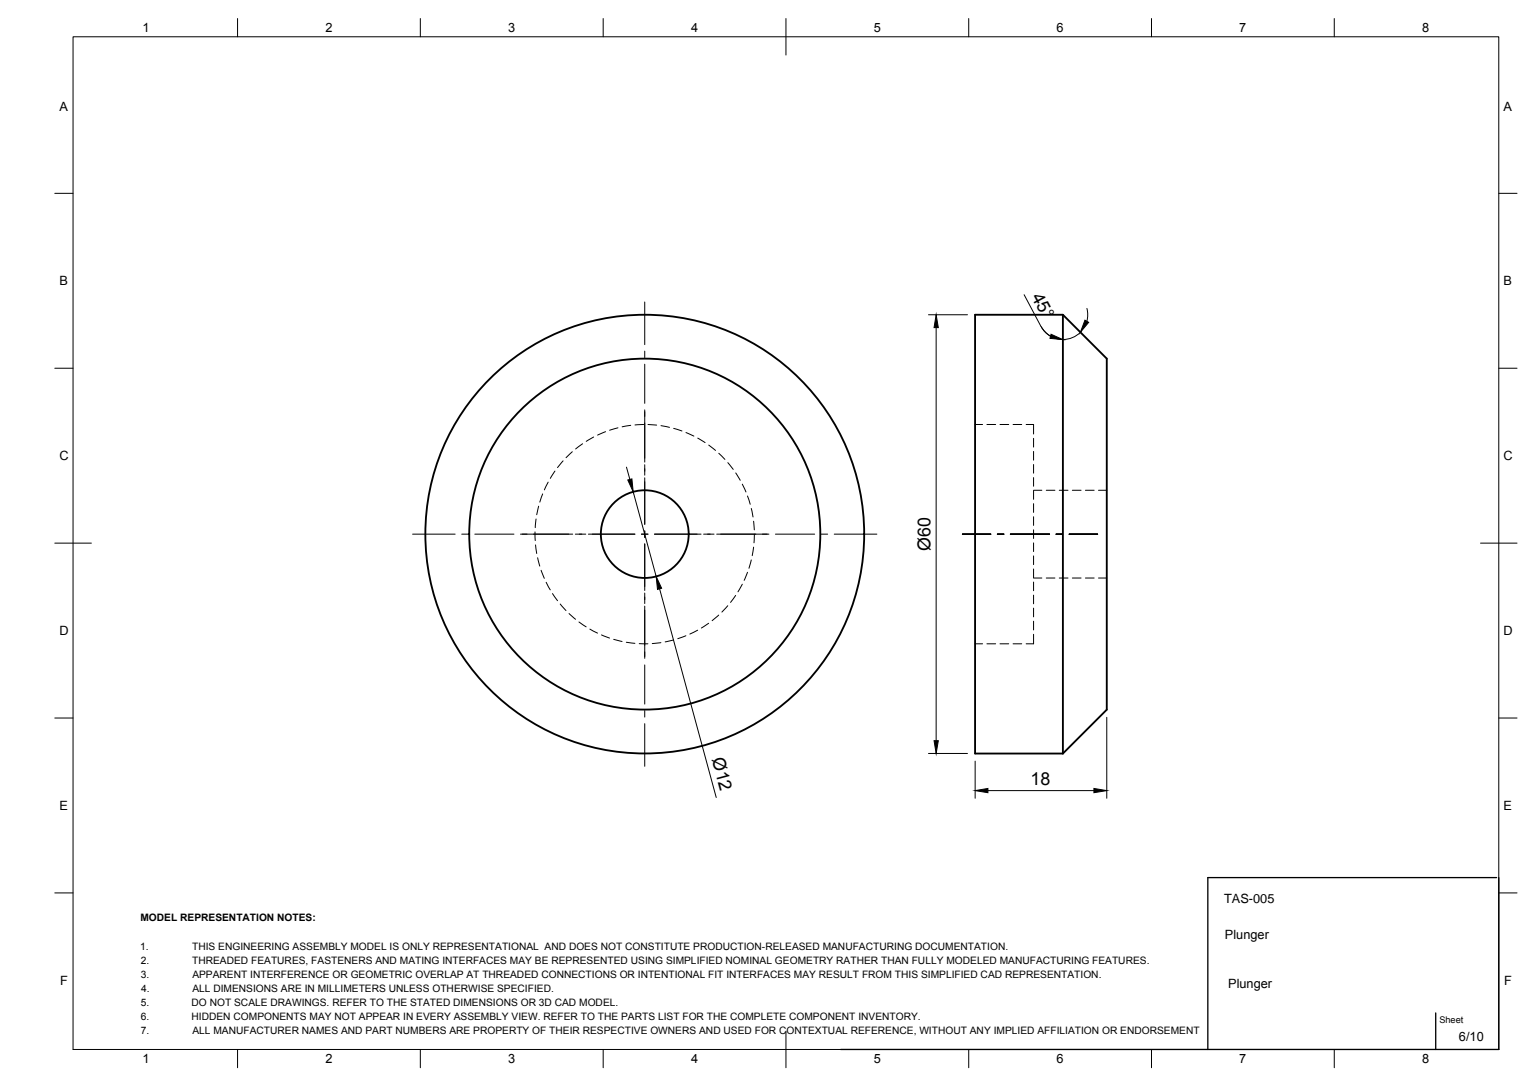
ISO-10303-21;
HEADER;
/* Generated by software containing ST-Developer
 * from STEP Tools, Inc. (www.steptools.com) 
 */

FILE_DESCRIPTION(
/* description */ ('STEP AP214'),
/* implementation_level */ '2;1');

FILE_NAME(
/* name */ 'plunger.step',
/* time_stamp */ '2026-11-04T19:54:22-08:00',
/* author */ (''),
/* organization */ (''),
/* preprocessor_version */ 'ST-DEVELOPER v20.2',
/* originating_system */ 'Autodesk Translation Framework v15.17.0.0',
/* authorisation */ '');

FILE_SCHEMA (('AUTOMOTIVE_DESIGN { 1 0 10303 214 3 1 1 }'));
ENDSEC;

DATA;
#10=MECHANICAL_DESIGN_GEOMETRIC_PRESENTATION_REPRESENTATION('',(#242),#14084);
#51=CONICAL_SURFACE('',#3729,30.,0.78539816339745);
#224=SHAPE_REPRESENTATION_RELATIONSHIP('SRR','None',#14123,#233);
#233=ADVANCED_BREP_SHAPE_REPRESENTATION('',(#251),#14078);
#242=STYLED_ITEM('',(#14175),#251);
#251=MANIFOLD_SOLID_BREP('Body1',#3468);
#267=FACE_BOUND('',#687,.T.);
#268=FACE_BOUND('',#689,.T.);
#269=FACE_BOUND('',#691,.T.);
#330=PLANE('',#3738);
#331=PLANE('',#3739);
#332=PLANE('',#3740);
#482=FACE_OUTER_BOUND('',#682,.T.);
#483=FACE_OUTER_BOUND('',#683,.T.);
#484=FACE_OUTER_BOUND('',#684,.T.);
#485=FACE_OUTER_BOUND('',#685,.T.);
#486=FACE_OUTER_BOUND('',#686,.T.);
#487=FACE_OUTER_BOUND('',#688,.T.);
#488=FACE_OUTER_BOUND('',#690,.T.);
#682=EDGE_LOOP('',(#2859,#2860,#2861,#2862));
#683=EDGE_LOOP('',(#2863,#2864,#2865,#2866,#2867));
#684=EDGE_LOOP('',(#2868,#2869,#2870,#2871,#2872));
#685=EDGE_LOOP('',(#2873,#2874,#2875,#2876));
#686=EDGE_LOOP('',(#2877));
#687=EDGE_LOOP('',(#2878));
#688=EDGE_LOOP('',(#2879));
#689=EDGE_LOOP('',(#2880));
#690=EDGE_LOOP('',(#2881));
#691=EDGE_LOOP('',(#2882));
#960=LINE('',#9192,#1217);
#961=LINE('',#9200,#1218);
#962=LINE('',#9204,#1219);
#963=LINE('',#9210,#1220);
#1217=VECTOR('',#4359,15.);
#1218=VECTOR('',#4368,30.);
#1219=VECTOR('',#4373,30.);
#1220=VECTOR('',#4380,6.);
#1319=CIRCLE('',#3727,15.);
#1320=CIRCLE('',#3728,15.);
#1321=CIRCLE('',#3730,30.);
#1322=CIRCLE('',#3731,30.);
#1323=CIRCLE('',#3732,24.);
#1324=CIRCLE('',#3734,30.);
#1325=CIRCLE('',#3736,6.);
#1326=CIRCLE('',#3737,6.);
#1597=VERTEX_POINT('',#9189);
#1598=VERTEX_POINT('',#9191);
#1599=VERTEX_POINT('',#9195);
#1600=VERTEX_POINT('',#9196);
#1601=VERTEX_POINT('',#9199);
#1602=VERTEX_POINT('',#9203);
#1603=VERTEX_POINT('',#9207);
#1604=VERTEX_POINT('',#9209);
#2033=EDGE_CURVE('',#1597,#1597,#1319,.T.);
#2034=EDGE_CURVE('',#1597,#1598,#960,.T.);
#2035=EDGE_CURVE('',#1598,#1598,#1320,.T.);
#2036=EDGE_CURVE('',#1599,#1600,#1321,.T.);
#2037=EDGE_CURVE('',#1600,#1599,#1322,.T.);
#2038=EDGE_CURVE('',#1600,#1601,#961,.T.);
#2039=EDGE_CURVE('',#1601,#1601,#1323,.T.);
#2040=EDGE_CURVE('',#1599,#1602,#962,.T.);
#2041=EDGE_CURVE('',#1602,#1602,#1324,.T.);
#2042=EDGE_CURVE('',#1603,#1603,#1325,.T.);
#2043=EDGE_CURVE('',#1603,#1604,#963,.T.);
#2044=EDGE_CURVE('',#1604,#1604,#1326,.T.);
#2859=ORIENTED_EDGE('',*,*,#2033,.F.);
#2860=ORIENTED_EDGE('',*,*,#2034,.T.);
#2861=ORIENTED_EDGE('',*,*,#2035,.T.);
#2862=ORIENTED_EDGE('',*,*,#2034,.F.);
#2863=ORIENTED_EDGE('',*,*,#2036,.F.);
#2864=ORIENTED_EDGE('',*,*,#2037,.F.);
#2865=ORIENTED_EDGE('',*,*,#2038,.T.);
#2866=ORIENTED_EDGE('',*,*,#2039,.F.);
#2867=ORIENTED_EDGE('',*,*,#2038,.F.);
#2868=ORIENTED_EDGE('',*,*,#2036,.T.);
#2869=ORIENTED_EDGE('',*,*,#2037,.T.);
#2870=ORIENTED_EDGE('',*,*,#2040,.T.);
#2871=ORIENTED_EDGE('',*,*,#2041,.F.);
#2872=ORIENTED_EDGE('',*,*,#2040,.F.);
#2873=ORIENTED_EDGE('',*,*,#2042,.T.);
#2874=ORIENTED_EDGE('',*,*,#2043,.T.);
#2875=ORIENTED_EDGE('',*,*,#2044,.F.);
#2876=ORIENTED_EDGE('',*,*,#2043,.F.);
#2877=ORIENTED_EDGE('',*,*,#2041,.T.);
#2878=ORIENTED_EDGE('',*,*,#2035,.F.);
#2879=ORIENTED_EDGE('',*,*,#2039,.T.);
#2880=ORIENTED_EDGE('',*,*,#2044,.T.);
#2881=ORIENTED_EDGE('',*,*,#2033,.T.);
#2882=ORIENTED_EDGE('',*,*,#2042,.F.);
#3256=CYLINDRICAL_SURFACE('',#3726,15.);
#3257=CYLINDRICAL_SURFACE('',#3733,30.);
#3258=CYLINDRICAL_SURFACE('',#3735,6.);
#3392=ADVANCED_FACE('',(#482),#3256,.F.);
#3393=ADVANCED_FACE('',(#483),#51,.T.);
#3394=ADVANCED_FACE('',(#484),#3257,.T.);
#3395=ADVANCED_FACE('',(#485),#3258,.F.);
#3396=ADVANCED_FACE('',(#486,#267),#330,.T.);
#3397=ADVANCED_FACE('',(#487,#268),#331,.F.);
#3398=ADVANCED_FACE('',(#488,#269),#332,.T.);
#3468=CLOSED_SHELL('',(#3392,#3393,#3394,#3395,#3396,#3397,#3398));
#3725=AXIS2_PLACEMENT_3D('',#9187,#4353,#4354);
#3726=AXIS2_PLACEMENT_3D('',#9188,#4355,#4356);
#3727=AXIS2_PLACEMENT_3D('',#9190,#4357,#4358);
#3728=AXIS2_PLACEMENT_3D('',#9193,#4360,#4361);
#3729=AXIS2_PLACEMENT_3D('',#9194,#4362,#4363);
#3730=AXIS2_PLACEMENT_3D('',#9197,#4364,#4365);
#3731=AXIS2_PLACEMENT_3D('',#9198,#4366,#4367);
#3732=AXIS2_PLACEMENT_3D('',#9201,#4369,#4370);
#3733=AXIS2_PLACEMENT_3D('',#9202,#4371,#4372);
#3734=AXIS2_PLACEMENT_3D('',#9205,#4374,#4375);
#3735=AXIS2_PLACEMENT_3D('',#9206,#4376,#4377);
#3736=AXIS2_PLACEMENT_3D('',#9208,#4378,#4379);
#3737=AXIS2_PLACEMENT_3D('',#9211,#4381,#4382);
#3738=AXIS2_PLACEMENT_3D('',#9212,#4383,#4384);
#3739=AXIS2_PLACEMENT_3D('',#9213,#4385,#4386);
#3740=AXIS2_PLACEMENT_3D('',#9214,#4387,#4388);
#4353=DIRECTION('axis',(0.,0.,1.));
#4354=DIRECTION('refdir',(1.,0.,0.));
#4355=DIRECTION('center_axis',(0.,-1.,0.));
#4356=DIRECTION('ref_axis',(0.,0.,-1.));
#4357=DIRECTION('center_axis',(0.,-1.,0.));
#4358=DIRECTION('ref_axis',(0.,0.,-1.));
#4359=DIRECTION('',(0.,-1.,0.));
#4360=DIRECTION('center_axis',(0.,-1.,0.));
#4361=DIRECTION('ref_axis',(0.,0.,-1.));
#4362=DIRECTION('center_axis',(0.,-1.,0.));
#4363=DIRECTION('ref_axis',(0.,0.,-1.));
#4364=DIRECTION('center_axis',(0.,-1.,0.));
#4365=DIRECTION('ref_axis',(0.,0.,-1.));
#4366=DIRECTION('center_axis',(0.,-1.,0.));
#4367=DIRECTION('ref_axis',(0.,0.,-1.));
#4368=DIRECTION('',(8.65956056235495E-17,0.707106781186546,-0.707106781186549));
#4369=DIRECTION('center_axis',(0.,1.,0.));
#4370=DIRECTION('ref_axis',(0.,0.,-1.));
#4371=DIRECTION('center_axis',(0.,1.,0.));
#4372=DIRECTION('ref_axis',(0.,0.,1.));
#4373=DIRECTION('',(0.,-1.,0.));
#4374=DIRECTION('center_axis',(0.,-1.,0.));
#4375=DIRECTION('ref_axis',(0.,0.,-1.));
#4376=DIRECTION('center_axis',(0.,1.,0.));
#4377=DIRECTION('ref_axis',(0.,0.,1.));
#4378=DIRECTION('center_axis',(0.,-1.,0.));
#4379=DIRECTION('ref_axis',(0.,0.,-1.));
#4380=DIRECTION('',(0.,1.,0.));
#4381=DIRECTION('center_axis',(0.,-1.,0.));
#4382=DIRECTION('ref_axis',(0.,0.,-1.));
#4383=DIRECTION('center_axis',(0.,-1.,0.));
#4384=DIRECTION('ref_axis',(0.,0.,-1.));
#4385=DIRECTION('center_axis',(0.,-1.,0.));
#4386=DIRECTION('ref_axis',(0.,0.,-1.));
#4387=DIRECTION('center_axis',(0.,-1.,0.));
#4388=DIRECTION('ref_axis',(0.,0.,-1.));
#9187=CARTESIAN_POINT('',(0.,0.,0.));
#9188=CARTESIAN_POINT('Origin',(0.,63.,0.));
#9189=CARTESIAN_POINT('',(-1.83697019872103E-15,63.,15.));
#9190=CARTESIAN_POINT('Origin',(0.,63.,0.));
#9191=CARTESIAN_POINT('',(-1.83697019872103E-15,55.,15.));
#9192=CARTESIAN_POINT('',(-1.83697019872103E-15,63.,15.));
#9193=CARTESIAN_POINT('Origin',(0.,55.,0.));
#9194=CARTESIAN_POINT('Origin',(0.,67.,0.));
#9195=CARTESIAN_POINT('',(3.67394039744206E-15,67.,-30.));
#9196=CARTESIAN_POINT('',(-3.67394039744206E-15,67.,30.));
#9197=CARTESIAN_POINT('Origin',(0.,67.,0.));
#9198=CARTESIAN_POINT('Origin',(0.,67.,0.));
#9199=CARTESIAN_POINT('',(-2.93915231795365E-15,73.,24.));
#9200=CARTESIAN_POINT('',(-3.67394039744206E-15,67.,30.));
#9201=CARTESIAN_POINT('Origin',(0.,73.,0.));
#9202=CARTESIAN_POINT('Origin',(0.,55.,0.));
#9203=CARTESIAN_POINT('',(-3.67394039744206E-15,55.,-30.));
#9204=CARTESIAN_POINT('',(-3.67394039744206E-15,55.,-30.));
#9205=CARTESIAN_POINT('Origin',(0.,55.,0.));
#9206=CARTESIAN_POINT('Origin',(0.,55.,0.));
#9207=CARTESIAN_POINT('',(-7.34788079488412E-16,63.,-6.));
#9208=CARTESIAN_POINT('Origin',(0.,63.,0.));
#9209=CARTESIAN_POINT('',(-7.34788079488412E-16,73.,-6.));
#9210=CARTESIAN_POINT('',(-7.34788079488412E-16,55.,-6.));
#9211=CARTESIAN_POINT('Origin',(0.,73.,0.));
#9212=CARTESIAN_POINT('Origin',(0.,55.,0.));
#9213=CARTESIAN_POINT('Origin',(0.,73.,0.));
#9214=CARTESIAN_POINT('Origin',(0.,63.,0.));
#14067=UNCERTAINTY_MEASURE_WITH_UNIT(LENGTH_MEASURE(0.01),#14085,
'DISTANCE_ACCURACY_VALUE',
'Maximum model space distance between geometric entities at asserted c
onnectivities');
#14073=UNCERTAINTY_MEASURE_WITH_UNIT(LENGTH_MEASURE(0.01),#14085,
'DISTANCE_ACCURACY_VALUE',
'Maximum model space distance between geometric entities at asserted c
onnectivities');
#14078=(
GEOMETRIC_REPRESENTATION_CONTEXT(3)
GLOBAL_UNCERTAINTY_ASSIGNED_CONTEXT((#14067))
GLOBAL_UNIT_ASSIGNED_CONTEXT((#14085,#14087,#14088))
REPRESENTATION_CONTEXT('','3D')
);
#14084=(
GEOMETRIC_REPRESENTATION_CONTEXT(3)
GLOBAL_UNCERTAINTY_ASSIGNED_CONTEXT((#14073))
GLOBAL_UNIT_ASSIGNED_CONTEXT((#14085,#14087,#14088))
REPRESENTATION_CONTEXT('','3D')
);
#14085=(
LENGTH_UNIT()
NAMED_UNIT(*)
SI_UNIT(.MILLI.,.METRE.)
);
#14087=(
NAMED_UNIT(*)
PLANE_ANGLE_UNIT()
SI_UNIT($,.RADIAN.)
);
#14088=(
NAMED_UNIT(*)
SI_UNIT($,.STERADIAN.)
SOLID_ANGLE_UNIT()
);
#14093=SHAPE_DEFINITION_REPRESENTATION(#14103,#14123);
#14103=PRODUCT_DEFINITION_SHAPE('',$,#14134);
#14123=SHAPE_REPRESENTATION('',(#3725),#14078);
#14129=PRODUCT_DEFINITION_CONTEXT('part definition',#14161,'design');
#14134=PRODUCT_DEFINITION('plunger','plunger',#14144,#14129);
#14144=PRODUCT_DEFINITION_FORMATION('',$,#14167);
#14161=APPLICATION_CONTEXT(
'Core Data for Automotive Mechanical Design Process');
#14162=PRODUCT_CONTEXT('part definition',#14161,'mechanical');
#14167=PRODUCT('plunger','plunger',$,(#14162));
#14175=PRESENTATION_STYLE_ASSIGNMENT((#14181));
#14181=SURFACE_STYLE_USAGE(.BOTH.,#14187);
#14187=SURFACE_SIDE_STYLE('',(#14193));
#14193=SURFACE_STYLE_FILL_AREA(#14199);
#14199=FILL_AREA_STYLE('Opaque(227,224,212)',(#14205));
#14205=FILL_AREA_STYLE_COLOUR('Opaque(227,224,212)',#14211);
#14211=COLOUR_RGB('Opaque(227,224,212)',0.890196078431372,0.87843137254902,
0.831372549019608);
ENDSEC;
END-ISO-10303-21;
